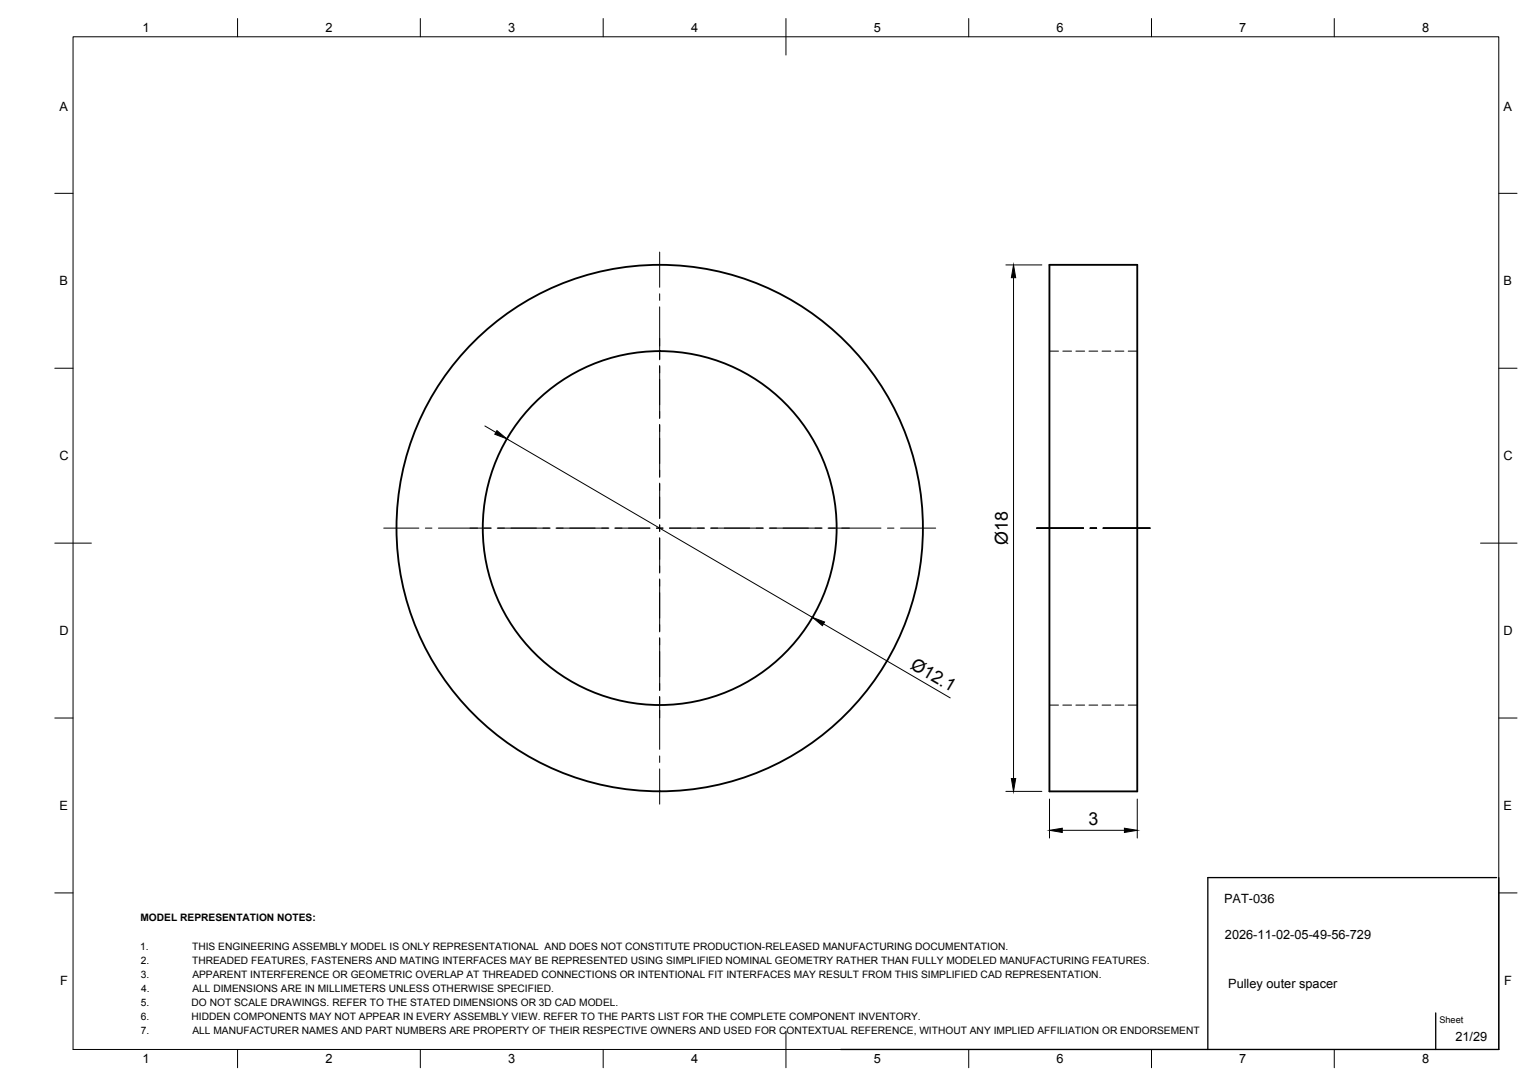
ISO-10303-21;
HEADER;
/* Generated by software containing ST-Developer
 * from STEP Tools, Inc. (www.steptools.com) 
 */

FILE_DESCRIPTION(
/* description */ ('Flange-mounted spindle'),
/* implementation_level */ '2;1');

FILE_NAME(
/* name */ 'Pulley outer spacer.step',
/* time_stamp */ '2026-10-27T10:49:51-07:00',
/* author */ (''),
/* organization */ (''),
/* preprocessor_version */ 'ST-DEVELOPER v20.2',
/* originating_system */ 'Autodesk Translation Framework v15.17.0.0',
/* authorisation */ '');

FILE_SCHEMA (('AUTOMOTIVE_DESIGN { 1 0 10303 214 3 1 1 }'));
ENDSEC;

DATA;
#10=MECHANICAL_DESIGN_GEOMETRIC_PRESENTATION_REPRESENTATION('',(#353),#11764);
#298=SHAPE_REPRESENTATION_RELATIONSHIP('SRR','None',#11896,#325);
#325=ADVANCED_BREP_SHAPE_REPRESENTATION('',(#379),#11751);
#353=STYLED_ITEM('',(#12085),#379);
#379=MANIFOLD_SOLID_BREP('Body1',#6147);
#459=FACE_BOUND('',#1234,.T.);
#460=FACE_BOUND('',#1236,.T.);
#596=PLANE('',#6723);
#597=PLANE('',#6724);
#818=FACE_OUTER_BOUND('',#1231,.T.);
#819=FACE_OUTER_BOUND('',#1232,.T.);
#820=FACE_OUTER_BOUND('',#1233,.T.);
#821=FACE_OUTER_BOUND('',#1235,.T.);
#1231=EDGE_LOOP('',(#4611,#4612,#4613,#4614));
#1232=EDGE_LOOP('',(#4615,#4616,#4617,#4618));
#1233=EDGE_LOOP('',(#4619));
#1234=EDGE_LOOP('',(#4620));
#1235=EDGE_LOOP('',(#4621));
#1236=EDGE_LOOP('',(#4622));
#1665=LINE('',#10215,#2087);
#1666=LINE('',#10221,#2088);
#2087=VECTOR('',#7914,0.605);
#2088=VECTOR('',#7921,0.9);
#2416=CIRCLE('',#6718,0.605);
#2417=CIRCLE('',#6719,0.605);
#2418=CIRCLE('',#6721,0.9);
#2419=CIRCLE('',#6722,0.9);
#2856=VERTEX_POINT('',#10212);
#2857=VERTEX_POINT('',#10214);
#2858=VERTEX_POINT('',#10218);
#2859=VERTEX_POINT('',#10220);
#3498=EDGE_CURVE('',#2856,#2856,#2416,.T.);
#3499=EDGE_CURVE('',#2856,#2857,#1665,.T.);
#3500=EDGE_CURVE('',#2857,#2857,#2417,.T.);
#3501=EDGE_CURVE('',#2858,#2858,#2418,.T.);
#3502=EDGE_CURVE('',#2858,#2859,#1666,.T.);
#3503=EDGE_CURVE('',#2859,#2859,#2419,.T.);
#4611=ORIENTED_EDGE('',*,*,#3498,.F.);
#4612=ORIENTED_EDGE('',*,*,#3499,.T.);
#4613=ORIENTED_EDGE('',*,*,#3500,.T.);
#4614=ORIENTED_EDGE('',*,*,#3499,.F.);
#4615=ORIENTED_EDGE('',*,*,#3501,.F.);
#4616=ORIENTED_EDGE('',*,*,#3502,.T.);
#4617=ORIENTED_EDGE('',*,*,#3503,.T.);
#4618=ORIENTED_EDGE('',*,*,#3502,.F.);
#4619=ORIENTED_EDGE('',*,*,#3501,.T.);
#4620=ORIENTED_EDGE('',*,*,#3498,.T.);
#4621=ORIENTED_EDGE('',*,*,#3503,.F.);
#4622=ORIENTED_EDGE('',*,*,#3500,.F.);
#5670=CYLINDRICAL_SURFACE('',#6717,0.605);
#5671=CYLINDRICAL_SURFACE('',#6720,0.9);
#5929=ADVANCED_FACE('',(#818),#5670,.F.);
#5930=ADVANCED_FACE('',(#819),#5671,.T.);
#5931=ADVANCED_FACE('',(#820,#459),#596,.T.);
#5932=ADVANCED_FACE('',(#821,#460),#597,.F.);
#6147=CLOSED_SHELL('',(#5929,#5930,#5931,#5932));
#6716=AXIS2_PLACEMENT_3D('',#10210,#7908,#7909);
#6717=AXIS2_PLACEMENT_3D('',#10211,#7910,#7911);
#6718=AXIS2_PLACEMENT_3D('',#10213,#7912,#7913);
#6719=AXIS2_PLACEMENT_3D('',#10216,#7915,#7916);
#6720=AXIS2_PLACEMENT_3D('',#10217,#7917,#7918);
#6721=AXIS2_PLACEMENT_3D('',#10219,#7919,#7920);
#6722=AXIS2_PLACEMENT_3D('',#10222,#7922,#7923);
#6723=AXIS2_PLACEMENT_3D('',#10223,#7924,#7925);
#6724=AXIS2_PLACEMENT_3D('',#10224,#7926,#7927);
#7908=DIRECTION('axis',(0.,0.,1.));
#7909=DIRECTION('refdir',(1.,0.,0.));
#7910=DIRECTION('center_axis',(0.,1.,0.));
#7911=DIRECTION('ref_axis',(1.,0.,0.));
#7912=DIRECTION('center_axis',(0.,-1.,0.));
#7913=DIRECTION('ref_axis',(1.,0.,0.));
#7914=DIRECTION('',(0.,-1.,0.));
#7915=DIRECTION('center_axis',(0.,-1.,0.));
#7916=DIRECTION('ref_axis',(1.,0.,0.));
#7917=DIRECTION('center_axis',(0.,1.,0.));
#7918=DIRECTION('ref_axis',(1.,0.,0.));
#7919=DIRECTION('center_axis',(0.,1.,0.));
#7920=DIRECTION('ref_axis',(1.,0.,0.));
#7921=DIRECTION('',(0.,-1.,0.));
#7922=DIRECTION('center_axis',(0.,1.,0.));
#7923=DIRECTION('ref_axis',(1.,0.,0.));
#7924=DIRECTION('center_axis',(0.,1.,0.));
#7925=DIRECTION('ref_axis',(1.,0.,0.));
#7926=DIRECTION('center_axis',(0.,1.,0.));
#7927=DIRECTION('ref_axis',(1.,0.,0.));
#10210=CARTESIAN_POINT('',(0.,0.,0.));
#10211=CARTESIAN_POINT('Origin',(0.,-7.,8.));
#10212=CARTESIAN_POINT('',(-0.605,-6.7,8.));
#10213=CARTESIAN_POINT('Origin',(0.,-6.7,8.));
#10214=CARTESIAN_POINT('',(-0.605,-7.,8.));
#10215=CARTESIAN_POINT('',(-0.605,-7.,8.));
#10216=CARTESIAN_POINT('Origin',(0.,-7.,8.));
#10217=CARTESIAN_POINT('Origin',(0.,-7.,8.));
#10218=CARTESIAN_POINT('',(-0.9,-6.7,8.));
#10219=CARTESIAN_POINT('Origin',(0.,-6.7,8.));
#10220=CARTESIAN_POINT('',(-0.9,-7.,8.));
#10221=CARTESIAN_POINT('',(-0.9,-7.,8.));
#10222=CARTESIAN_POINT('Origin',(0.,-7.,8.));
#10223=CARTESIAN_POINT('Origin',(0.,-6.7,8.));
#10224=CARTESIAN_POINT('Origin',(0.,-7.,8.));
#11719=UNCERTAINTY_MEASURE_WITH_UNIT(LENGTH_MEASURE(0.001),#11765,
'DISTANCE_ACCURACY_VALUE',
'Maximum model space distance between geometric entities at asserted c
onnectivities');
#11732=UNCERTAINTY_MEASURE_WITH_UNIT(LENGTH_MEASURE(0.001),#11765,
'DISTANCE_ACCURACY_VALUE',
'Maximum model space distance between geometric entities at asserted c
onnectivities');
#11751=(
GEOMETRIC_REPRESENTATION_CONTEXT(3)
GLOBAL_UNCERTAINTY_ASSIGNED_CONTEXT((#11719))
GLOBAL_UNIT_ASSIGNED_CONTEXT((#11765,#11767,#11768))
REPRESENTATION_CONTEXT('','3D')
);
#11764=(
GEOMETRIC_REPRESENTATION_CONTEXT(3)
GLOBAL_UNCERTAINTY_ASSIGNED_CONTEXT((#11732))
GLOBAL_UNIT_ASSIGNED_CONTEXT((#11765,#11767,#11768))
REPRESENTATION_CONTEXT('','3D')
);
#11765=(
LENGTH_UNIT()
NAMED_UNIT(*)
SI_UNIT(.CENTI.,.METRE.)
);
#11767=(
NAMED_UNIT(*)
PLANE_ANGLE_UNIT()
SI_UNIT($,.RADIAN.)
);
#11768=(
NAMED_UNIT(*)
SI_UNIT($,.STERADIAN.)
SOLID_ANGLE_UNIT()
);
#11787=SHAPE_DEFINITION_REPRESENTATION(#11820,#11896);
#11820=PRODUCT_DEFINITION_SHAPE('',$,#11928);
#11896=SHAPE_REPRESENTATION('',(#6716),#11751);
#11909=PRODUCT_DEFINITION_CONTEXT('part definition',#12004,'design');
#11928=PRODUCT_DEFINITION('Pulley outer spacer','Pulley outer spacer',#11959,
#11909);
#11959=PRODUCT_DEFINITION_FORMATION('',$,#12024);
#12004=APPLICATION_CONTEXT(
'Core Data for Automotive Mechanical Design Process');
#12005=PRODUCT_CONTEXT('part definition',#12004,'mechanical');
#12024=PRODUCT('Pulley outer spacer','Pulley outer spacer',
'Pulley outer spacer',(#12005));
#12079=COLOUR_RGB('Light Blue',0.38,0.62,0.78);
#12080=FILL_AREA_STYLE_COLOUR('',#12079);
#12081=FILL_AREA_STYLE('',(#12080));
#12082=SURFACE_STYLE_FILL_AREA(#12081);
#12083=SURFACE_SIDE_STYLE('',(#12082));
#12084=SURFACE_STYLE_USAGE(.BOTH.,#12083);
#12085=PRESENTATION_STYLE_ASSIGNMENT((#12084));
ENDSEC;
END-ISO-10303-21;
